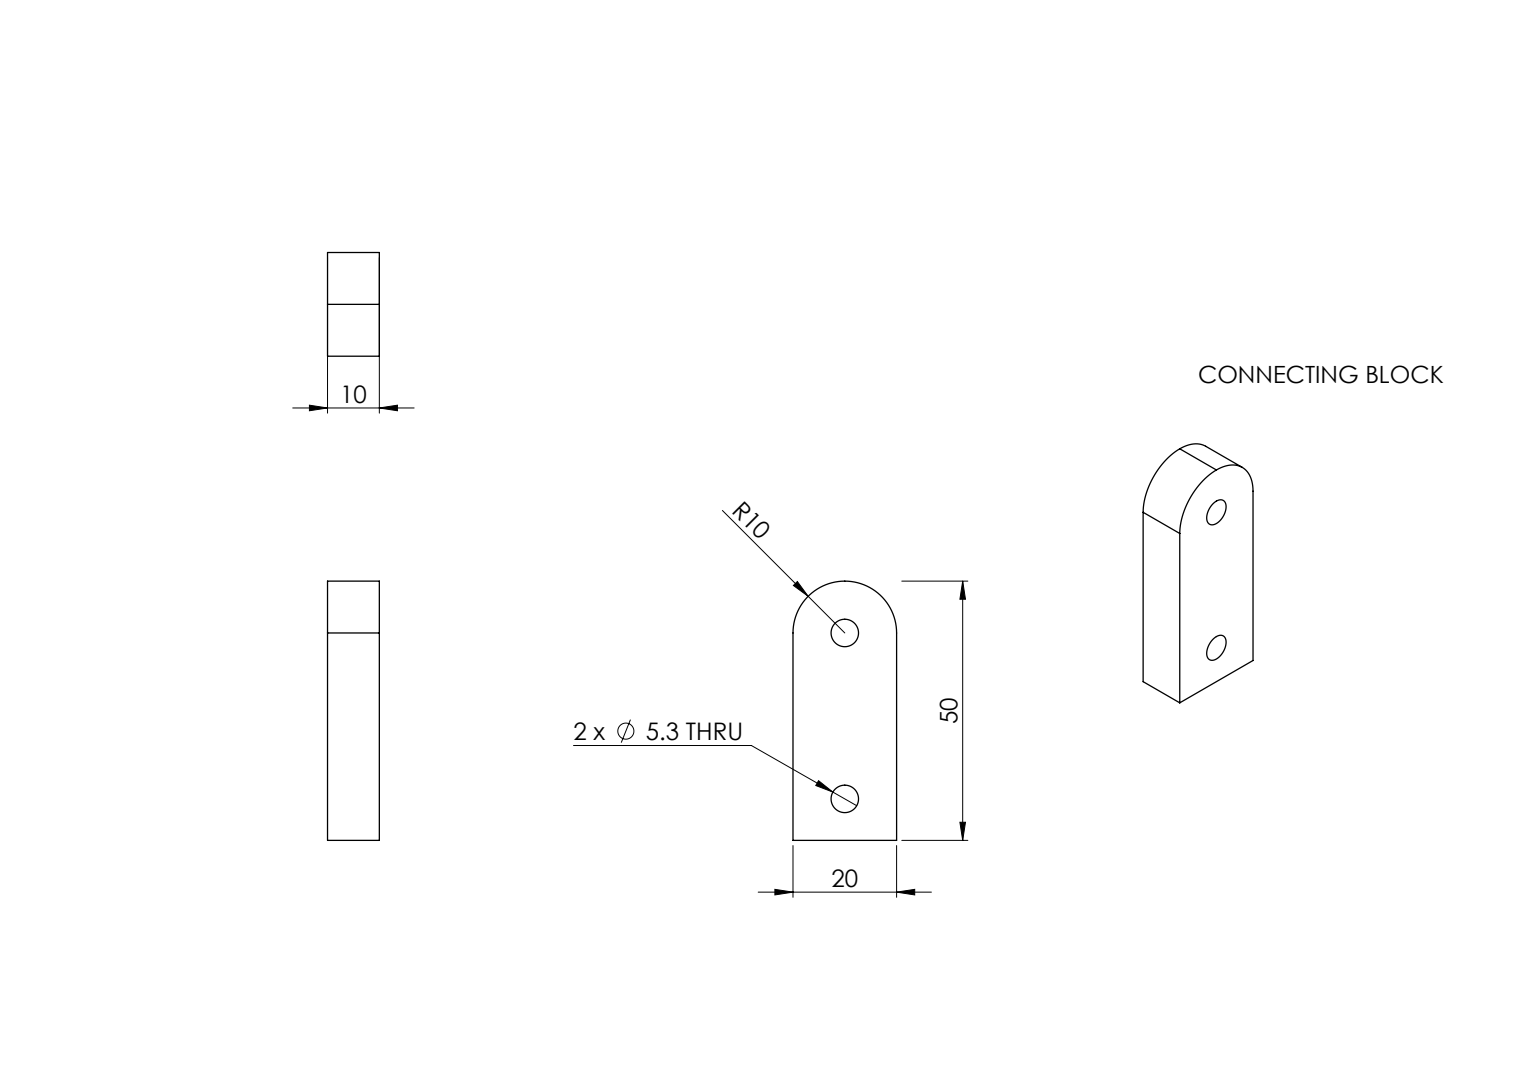
ISO-10303-21;
HEADER;
FILE_DESCRIPTION (('STEP AP214'),
    '1' );
FILE_NAME ('connecting block.step',
    '2026-10-25T17:17:34',
    ( '' ),
    ( '' ),
    'SwSTEP 2.0',
    'SolidWorks 2026',
    '' );
FILE_SCHEMA (( 'AUTOMOTIVE_DESIGN' ));
ENDSEC;

DATA;
#66=PLANE ( 'NONE',  #10236 ) ;
#158=DIRECTION ( 'NONE',  ( 0.000000000000000000, 1.000000000000000000, 0.000000000000000000 ) ) ;
#180=CARTESIAN_POINT ( 'NONE',  ( 109.9999999999999432, -29.80000000000002558, -150.0000000000000000 ) ) ;
#210=CARTESIAN_POINT ( 'NONE',  ( 99.99999999999994316, -29.80000000000000782, -150.0000000000000000 ) ) ;
#223=SHAPE_REPRESENTATION_RELATIONSHIP ( 'NONE' , 'NONE' ,  #14995, #14131 ) ;
#313=DIRECTION ( 'NONE',  ( 1.000000000000000000, -1.387778780781445676E-15, -2.407412430484046130E-31 ) ) ;
#489=CARTESIAN_POINT ( 'NONE',  ( 110.0000000000000142, 20.19999999999997797, -140.0000000000000000 ) ) ;
#517=ORIENTED_EDGE ( 'NONE', *, *, #5469, .F. ) ;
#541=CARTESIAN_POINT ( 'NONE',  ( 109.9999999999999574, -21.80000000000003268, -139.9999999999999716 ) ) ;
#670=ORIENTED_EDGE ( 'NONE', *, *, #8877, .T. ) ;
#820=AXIS2_PLACEMENT_3D ( 'NONE', #14217, #14502, #3869 ) ;
#918=DIRECTION ( 'NONE',  ( 1.000000000000000000, -0.000000000000000000, -2.407412430484046130E-31 ) ) ;
#945=EDGE_CURVE ( 'NONE', #2644, #11697, #6762, .T. ) ;
#972=ORIENTED_EDGE ( 'NONE', *, *, #12588, .F. ) ;
#1043=CLOSED_SHELL ( 'NONE', ( #15727, #1878, #15369, #14233, #4639, #15697, #12649, #17613, #16169, #5440, #19146 ) ) ;
#1064=ORIENTED_EDGE ( 'NONE', *, *, #3609, .F. ) ;
#1096=ORIENTED_EDGE ( 'NONE', *, *, #11672, .F. ) ;
#1137=CARTESIAN_POINT ( 'NONE',  ( 100.0000000000000000, 10.19999999999999396, -130.0000000000000000 ) ) ;
#1191=( GEOMETRIC_REPRESENTATION_CONTEXT ( 3 ) GLOBAL_UNCERTAINTY_ASSIGNED_CONTEXT ( ( #18445 ) ) GLOBAL_UNIT_ASSIGNED_CONTEXT ( ( #14859, #13397, #18984 ) ) REPRESENTATION_CONTEXT ( 'NONE', 'WORKASPACE' ) );
#1244=CARTESIAN_POINT ( 'NONE',  ( 110.0000000000000000, 10.19999999999997620, -139.9999999999999716 ) ) ;
#1398=ORIENTED_EDGE ( 'NONE', *, *, #4541, .F. ) ;
#1486=( NAMED_UNIT ( * ) PLANE_ANGLE_UNIT ( ) SI_UNIT ( $, .RADIAN. ) );
#1508=AXIS2_PLACEMENT_3D ( 'NONE', #9648, #2018, #10720 ) ;
#1521=ORIENTED_EDGE ( 'NONE', *, *, #7205, .T. ) ;
#1575=FACE_BOUND ( 'NONE', #12964, .T. ) ;
#1616=DIRECTION ( 'NONE',  ( 1.000000000000000000, -0.000000000000000000, -2.407412430484046130E-31 ) ) ;
#1660=ORIENTED_EDGE ( 'NONE', *, *, #11468, .T. ) ;
#1667=DIRECTION ( 'NONE',  ( -0.000000000000000000, 3.469446951953616161E-16, -1.000000000000000000 ) ) ;
#1747=CARTESIAN_POINT ( 'NONE',  ( 100.0000000000000000, 10.19999999999999218, -140.0000000000000000 ) ) ;
#1756=FACE_OUTER_BOUND ( 'NONE', #9533, .T. ) ;
#1775=EDGE_LOOP ( 'NONE', ( #3436, #14144, #6656, #3600 ) ) ;
#1829=ORIENTED_EDGE ( 'NONE', *, *, #5453, .T. ) ;
#1878=ADVANCED_FACE ( 'NONE', ( #10493 ), #15082, .F. ) ;
#1941=CARTESIAN_POINT ( 'NONE',  ( 100.0000000000000000, 10.19999999999997620, -142.6499999999999773 ) ) ;
#1993=ORIENTED_EDGE ( 'NONE', *, *, #4541, .T. ) ;
#2018=DIRECTION ( 'NONE',  ( 1.000000000000000000, -1.387778780781445676E-15, -2.407412430484046130E-31 ) ) ;
#2029=PRODUCT_CONTEXT ( 'NONE', #3323, 'mechanical' ) ;
#2039=EDGE_CURVE ( 'NONE', #3376, #2644, #2875, .T. ) ;
#2055=EDGE_LOOP ( 'NONE', ( #11819, #10542, #1398, #11442 ) ) ;
#2149=CARTESIAN_POINT ( 'NONE',  ( 110.0000000000000000, 10.19999999999997620, -150.0000000000000000 ) ) ;
#2320=EDGE_CURVE ( 'NONE', #17568, #9852, #15512, .T. ) ;
#2364=VECTOR ( 'NONE', #12931, 1000.000000000000000 ) ;
#2381=CARTESIAN_POINT ( 'NONE',  ( 110.0000000000000000, 10.19999999999997620, -139.9999999999999716 ) ) ;
#2411=CYLINDRICAL_SURFACE ( 'NONE', #16456, 10.00000000000000000 ) ;
#2569=DIRECTION ( 'NONE',  ( 1.000000000000000000, -1.387778780781445676E-15, -2.407412430484046130E-31 ) ) ;
#2628=ORIENTED_EDGE ( 'NONE', *, *, #2320, .F. ) ;
#2644=VERTEX_POINT ( 'NONE', #19175 ) ;
#2645=( NAMED_UNIT ( * ) SI_UNIT ( $, .STERADIAN. ) SOLID_ANGLE_UNIT ( ) );
#2685=LINE ( 'NONE', #9930, #9733 ) ;
#2706=LINE ( 'NONE', #180, #17740 ) ;
#2828=EDGE_CURVE ( 'NONE', #14354, #11020, #7827, .T. ) ;
#2875=LINE ( 'NONE', #6004, #5398 ) ;
#2934=DIRECTION ( 'NONE',  ( 1.000000000000000000, -1.387778780781445676E-15, -2.407412430484046130E-31 ) ) ;
#2998=DIRECTION ( 'NONE',  ( 0.000000000000000000, 1.000000000000000000, 0.000000000000000000 ) ) ;
#3041=CARTESIAN_POINT ( 'NONE',  ( 109.9999999999999432, -29.80000000000003268, -130.0000000000000000 ) ) ;
#3081=CYLINDRICAL_SURFACE ( 'NONE', #17126, 2.649999999999985700 ) ;
#3084=VERTEX_POINT ( 'NONE', #6227 ) ;
#3104=FACE_OUTER_BOUND ( 'NONE', #2055, .T. ) ;
#3218=CARTESIAN_POINT ( 'NONE',  ( 99.99999999999998579, -1.387778780781445676E-13, -2.407412430484045937E-29 ) ) ;
#3253=DIRECTION ( 'NONE',  ( -0.000000000000000000, 3.469446951953616161E-16, -1.000000000000000000 ) ) ;
#3323=APPLICATION_CONTEXT ( 'automotive_design' ) ;
#3325=DIRECTION ( 'NONE',  ( 0.000000000000000000, 1.000000000000000000, 0.000000000000000000 ) ) ;
#3359=CARTESIAN_POINT ( 'NONE',  ( 109.9999999999999432, -29.80000000000003268, -130.0000000000000000 ) ) ;
#3376=VERTEX_POINT ( 'NONE', #3041 ) ;
#3395=CARTESIAN_POINT ( 'NONE',  ( 109.9999999999999574, -21.80000000000003268, -137.3499999999999943 ) ) ;
#3429=ORIENTED_EDGE ( 'NONE', *, *, #16643, .F. ) ;
#3436=ORIENTED_EDGE ( 'NONE', *, *, #7205, .F. ) ;
#3474=ORIENTED_EDGE ( 'NONE', *, *, #2828, .T. ) ;
#3484=CARTESIAN_POINT ( 'NONE',  ( 99.99999999999994316, -29.80000000000000782, -150.0000000000000000 ) ) ;
#3507=AXIS2_PLACEMENT_3D ( 'NONE', #9368, #313, #6452 ) ;
#3600=ORIENTED_EDGE ( 'NONE', *, *, #4576, .F. ) ;
#3609=EDGE_CURVE ( 'NONE', #6906, #6376, #16464, .T. ) ;
#3618=VECTOR ( 'NONE', #8272, 1000.000000000000000 ) ;
#3669=CARTESIAN_POINT ( 'NONE',  ( 110.9999999999999574, -21.80000000000003268, -142.6499999999999773 ) ) ;
#3791=ORIENTED_EDGE ( 'NONE', *, *, #4723, .T. ) ;
#3869=DIRECTION ( 'NONE',  ( 1.387778780781445676E-15, 1.000000000000000000, -2.775557561562891351E-15 ) ) ;
#3999=AXIS2_PLACEMENT_3D ( 'NONE', #16398, #4385, #16215 ) ;
#4087=CARTESIAN_POINT ( 'NONE',  ( 100.0000000000000000, 10.19999999999997620, -139.9999999999999716 ) ) ;
#4203=LINE ( 'NONE', #10070, #8822 ) ;
#4346=DIRECTION ( 'NONE',  ( 1.000000000000000000, -0.000000000000000000, -2.407412430484046130E-31 ) ) ;
#4357=FACE_OUTER_BOUND ( 'NONE', #7999, .T. ) ;
#4375=CARTESIAN_POINT ( 'NONE',  ( 100.0000000000000000, 10.19999999999997620, -137.3499999999999943 ) ) ;
#4385=DIRECTION ( 'NONE',  ( -1.000000000000000000, 1.586032892321652482E-15, 0.000000000000000000 ) ) ;
#4413=PRESENTATION_STYLE_ASSIGNMENT (( #8611 ) ) ;
#4465=EDGE_CURVE ( 'NONE', #11020, #7039, #13361, .T. ) ;
#4538=ORIENTED_EDGE ( 'NONE', *, *, #8760, .F. ) ;
#4541=EDGE_CURVE ( 'NONE', #7039, #11136, #12486, .T. ) ;
#4542=CIRCLE ( 'NONE', #10784, 2.649999999999980371 ) ;
#4576=EDGE_CURVE ( 'NONE', #5794, #6376, #4790, .T. ) ;
#4639=ADVANCED_FACE ( 'NONE', ( #18652 ), #15907, .F. ) ;
#4653=DIRECTION ( 'NONE',  ( 0.000000000000000000, 0.000000000000000000, -1.000000000000000000 ) ) ;
#4723=EDGE_CURVE ( 'NONE', #2644, #7081, #2706, .T. ) ;
#4765=VECTOR ( 'NONE', #14074, 1000.000000000000000 ) ;
#4790=LINE ( 'NONE', #6442, #13665 ) ;
#4794=CIRCLE ( 'NONE', #7888, 9.999999999999998224 ) ;
#4841=CARTESIAN_POINT ( 'NONE',  ( 110.9999999999999574, -21.80000000000003268, -139.9999999999999716 ) ) ;
#4895=DIRECTION ( 'NONE',  ( 1.387778780781445873E-15, 1.000000000000000000, 0.000000000000000000 ) ) ;
#4936=LINE ( 'NONE', #3359, #5998 ) ;
#4993=CARTESIAN_POINT ( 'NONE',  ( 100.0000000000000000, 10.19999999999997620, -139.9999999999999716 ) ) ;
#5099=EDGE_LOOP ( 'NONE', ( #4538, #17421, #7613, #1660 ) ) ;
#5232=AXIS2_PLACEMENT_3D ( 'NONE', #6966, #9796, #18700 ) ;
#5276=VERTEX_POINT ( 'NONE', #10120 ) ;
#5316=FACE_OUTER_BOUND ( 'NONE', #1775, .T. ) ;
#5398=VECTOR ( 'NONE', #3253, 1000.000000000000000 ) ;
#5440=ADVANCED_FACE ( 'NONE', ( #12445 ), #16746, .F. ) ;
#5453=EDGE_CURVE ( 'NONE', #8145, #9264, #12430, .T. ) ;
#5469=EDGE_CURVE ( 'NONE', #14354, #3376, #4936, .T. ) ;
#5508=FACE_OUTER_BOUND ( 'NONE', #8430, .T. ) ;
#5560=( GEOMETRIC_REPRESENTATION_CONTEXT ( 3 ) GLOBAL_UNCERTAINTY_ASSIGNED_CONTEXT ( ( #13232 ) ) GLOBAL_UNIT_ASSIGNED_CONTEXT ( ( #17901, #1486, #2645 ) ) REPRESENTATION_CONTEXT ( 'NONE', 'WORKASPACE' ) );
#5570=AXIS2_PLACEMENT_3D ( 'NONE', #17281, #9661, #12969 ) ;
#5577=CIRCLE ( 'NONE', #1508, 9.999999999999998224 ) ;
#5683=CARTESIAN_POINT ( 'NONE',  ( 111.0000000000000000, 10.19999999999997620, -137.3499999999999943 ) ) ;
#5736=DIRECTION ( 'NONE',  ( -0.000000000000000000, 0.000000000000000000, 1.000000000000000000 ) ) ;
#5768=DIRECTION ( 'NONE',  ( 1.000000000000000000, -0.000000000000000000, -2.407412430484046130E-31 ) ) ;
#5784=FILL_AREA_STYLE ('',( #17803 ) ) ;
#5794=VERTEX_POINT ( 'NONE', #1941 ) ;
#5899=DIRECTION ( 'NONE',  ( 1.000000000000000000, -1.387778780781445676E-15, -2.407412430484046130E-31 ) ) ;
#5998=VECTOR ( 'NONE', #16851, 1000.000000000000000 ) ;
#6004=CARTESIAN_POINT ( 'NONE',  ( 109.9999999999999432, -29.80000000000002558, -150.0000000000000000 ) ) ;
#6010=CIRCLE ( 'NONE', #3507, 2.649999999999982148 ) ;
#6028=VECTOR ( 'NONE', #5768, 1000.000000000000000 ) ;
#6188=VERTEX_POINT ( 'NONE', #4375 ) ;
#6227=CARTESIAN_POINT ( 'NONE',  ( 100.0000000000000000, 10.19999999999999396, -150.0000000000000000 ) ) ;
#6359=CARTESIAN_POINT ( 'NONE',  ( 110.0000000000000000, 10.19999999999997620, -139.9999999999999716 ) ) ;
#6369=EDGE_LOOP ( 'NONE', ( #17719, #15739, #15622, #12797 ) ) ;
#6370=DIRECTION ( 'NONE',  ( -1.000000000000000000, 1.586032892321652482E-15, 0.000000000000000000 ) ) ;
#6376=VERTEX_POINT ( 'NONE', #16677 ) ;
#6442=CARTESIAN_POINT ( 'NONE',  ( 111.0000000000000000, 10.19999999999997620, -142.6499999999999773 ) ) ;
#6452=DIRECTION ( 'NONE',  ( 0.000000000000000000, 1.000000000000000000, 0.000000000000000000 ) ) ;
#6616=EDGE_CURVE ( 'NONE', #11697, #3084, #2685, .T. ) ;
#6648=CARTESIAN_POINT ( 'NONE',  ( 100.0000000000000142, 20.19999999999999574, -140.0000000000000000 ) ) ;
#6656=ORIENTED_EDGE ( 'NONE', *, *, #3609, .T. ) ;
#6659=DIRECTION ( 'NONE',  ( 1.000000000000000000, -1.387778780781445676E-15, -2.407412430484046130E-31 ) ) ;
#6681=PLANE ( 'NONE',  #5232 ) ;
#6762=LINE ( 'NONE', #15839, #4765 ) ;
#6802=COLOUR_RGB ( '',0.8941176470588234615, 0.8941176470588234615, 0.8941176470588234615 ) ;
#6906=VERTEX_POINT ( 'NONE', #19184 ) ;
#6966=CARTESIAN_POINT ( 'NONE',  ( 109.9999999999999858, -1.546382070013610932E-13, -2.407412430484045937E-29 ) ) ;
#7013=EDGE_CURVE ( 'NONE', #9852, #17568, #6010, .T. ) ;
#7039=VERTEX_POINT ( 'NONE', #6648 ) ;
#7081=VERTEX_POINT ( 'NONE', #2149 ) ;
#7106=ORIENTED_EDGE ( 'NONE', *, *, #11374, .F. ) ;
#7111=STYLED_ITEM ( 'NONE', ( #4413 ), #14131 ) ;
#7205=EDGE_CURVE ( 'NONE', #6188, #5794, #10689, .T. ) ;
#7262=AXIS2_PLACEMENT_3D ( 'NONE', #4993, #10936, #15431 ) ;
#7264=CARTESIAN_POINT ( 'NONE',  ( 110.0000000000000000, 10.19999999999997620, -130.0000000000000000 ) ) ;
#7327=ORIENTED_EDGE ( 'NONE', *, *, #2039, .T. ) ;
#7341=CARTESIAN_POINT ( 'NONE',  ( 0.000000000000000000, 0.000000000000000000, 0.000000000000000000 ) ) ;
#7516=MANIFOLD_SOLID_BREP ( 'M5 Clearance Hole1', #1043 ) ;
#7523=DIRECTION ( 'NONE',  ( 1.387778780781445676E-15, 1.000000000000000000, 0.000000000000000000 ) ) ;
#7578=DIRECTION ( 'NONE',  ( 0.000000000000000000, 0.000000000000000000, -1.000000000000000000 ) ) ;
#7613=ORIENTED_EDGE ( 'NONE', *, *, #4576, .T. ) ;
#7827=LINE ( 'NONE', #13782, #8641 ) ;
#7888=AXIS2_PLACEMENT_3D ( 'NONE', #6359, #15634, #4895 ) ;
#7932=EDGE_CURVE ( 'NONE', #7081, #11136, #4794, .T. ) ;
#7999=EDGE_LOOP ( 'NONE', ( #517, #3474, #11002, #14020 ) ) ;
#8145=VERTEX_POINT ( 'NONE', #3395 ) ;
#8272=DIRECTION ( 'NONE',  ( 1.000000000000000000, -1.586032892321652482E-15, 0.000000000000000000 ) ) ;
#8359=EDGE_LOOP ( 'NONE', ( #2628, #12481, #1829, #3429 ) ) ;
#8430=EDGE_LOOP ( 'NONE', ( #3791, #12729, #15733, #8546, #7327 ) ) ;
#8435=CARTESIAN_POINT ( 'NONE',  ( 110.9999999999999574, -21.80000000000003268, -137.3499999999999943 ) ) ;
#8463=FACE_OUTER_BOUND ( 'NONE', #12711, .T. ) ;
#8546=ORIENTED_EDGE ( 'NONE', *, *, #5469, .T. ) ;
#8593=ORIENTED_EDGE ( 'NONE', *, *, #7013, .T. ) ;
#8611=SURFACE_STYLE_USAGE ( .BOTH. , #10281 ) ;
#8641=VECTOR ( 'NONE', #6370, 1000.000000000000000 ) ;
#8654=CARTESIAN_POINT ( 'NONE',  ( 111.0000000000000000, 10.19999999999997620, -139.9999999999999716 ) ) ;
#8696=LINE ( 'NONE', #5683, #6028 ) ;
#8760=EDGE_CURVE ( 'NONE', #6188, #6906, #8696, .T. ) ;
#8817=CARTESIAN_POINT ( 'NONE',  ( 109.9999999999999574, -21.80000000000003268, -139.9999999999999716 ) ) ;
#8822=VECTOR ( 'NONE', #13277, 1000.000000000000000 ) ;
#8877=EDGE_CURVE ( 'NONE', #3376, #5276, #4203, .T. ) ;
#9040=DIRECTION ( 'NONE',  ( 1.000000000000000000, 0.000000000000000000, 0.000000000000000000 ) ) ;
#9098=EDGE_CURVE ( 'NONE', #9264, #8145, #10085, .T. ) ;
#9264=VERTEX_POINT ( 'NONE', #9488 ) ;
#9368=CARTESIAN_POINT ( 'NONE',  ( 99.99999999999995737, -21.80000000000003268, -139.9999999999999716 ) ) ;
#9480=ORIENTED_EDGE ( 'NONE', *, *, #2039, .F. ) ;
#9488=CARTESIAN_POINT ( 'NONE',  ( 109.9999999999999574, -21.80000000000003268, -142.6499999999999773 ) ) ;
#9533=EDGE_LOOP ( 'NONE', ( #16683, #13175, #14475, #972, #9819 ) ) ;
#9648=CARTESIAN_POINT ( 'NONE',  ( 110.0000000000000000, 10.19999999999997620, -140.0000000000000000 ) ) ;
#9661=DIRECTION ( 'NONE',  ( 1.586032892321652482E-15, 1.000000000000000000, 3.469446951953616654E-16 ) ) ;
#9733=VECTOR ( 'NONE', #11489, 1000.000000000000000 ) ;
#9796=DIRECTION ( 'NONE',  ( 1.000000000000000000, -1.387778780781445676E-15, -2.407412430484046130E-31 ) ) ;
#9819=ORIENTED_EDGE ( 'NONE', *, *, #15245, .F. ) ;
#9852=VERTEX_POINT ( 'NONE', #16105 ) ;
#9884=EDGE_CURVE ( 'NONE', #5794, #6188, #16382, .T. ) ;
#9930=CARTESIAN_POINT ( 'NONE',  ( 99.99999999999994316, -29.80000000000000782, -150.0000000000000000 ) ) ;
#9934=AXIS2_PLACEMENT_3D ( 'NONE', #1747, #15229, #15321 ) ;
#9988=( NAMED_UNIT ( * ) PLANE_ANGLE_UNIT ( ) SI_UNIT ( $, .RADIAN. ) );
#10033=CARTESIAN_POINT ( 'NONE',  ( 99.99999999999994316, -29.80000000000001492, -130.0000000000000000 ) ) ;
#10070=CARTESIAN_POINT ( 'NONE',  ( 109.9999999999999432, -29.80000000000003268, -130.0000000000000000 ) ) ;
#10085=CIRCLE ( 'NONE', #12573, 2.649999999999982148 ) ;
#10120=CARTESIAN_POINT ( 'NONE',  ( 99.99999999999994316, -29.80000000000001492, -130.0000000000000000 ) ) ;
#10130=FACE_OUTER_BOUND ( 'NONE', #6369, .T. ) ;
#10156=ORIENTED_EDGE ( 'NONE', *, *, #9098, .F. ) ;
#10236=AXIS2_PLACEMENT_3D ( 'NONE', #15001, #4653, #16471 ) ;
#10281=SURFACE_SIDE_STYLE ('',( #17705 ) ) ;
#10359=LINE ( 'NONE', #210, #18915 ) ;
#10373=MECHANICAL_DESIGN_GEOMETRIC_PRESENTATION_REPRESENTATION('',(#18805),#17871);
#10476=DIRECTION ( 'NONE',  ( 0.000000000000000000, 1.000000000000000000, 0.000000000000000000 ) ) ;
#10493=FACE_OUTER_BOUND ( 'NONE', #8359, .T. ) ;
#10509=FACE_OUTER_BOUND ( 'NONE', #5099, .T. ) ;
#10514=AXIS2_PLACEMENT_3D ( 'NONE', #14565, #17609, #17228 ) ;
#10529=AXIS2_PLACEMENT_3D ( 'NONE', #11135, #6659, #3325 ) ;
#10540=AXIS2_PLACEMENT_3D ( 'NONE', #7341, #19270, #11738 ) ;
#10542=ORIENTED_EDGE ( 'NONE', *, *, #13895, .F. ) ;
#10689=CIRCLE ( 'NONE', #7262, 2.649999999999980371 ) ;
#10720=DIRECTION ( 'NONE',  ( 1.387778780781445873E-15, 1.000000000000000000, 0.000000000000000000 ) ) ;
#10784=AXIS2_PLACEMENT_3D ( 'NONE', #2381, #2569, #11270 ) ;
#10900=EDGE_CURVE ( 'NONE', #7039, #3084, #18287, .T. ) ;
#10936=DIRECTION ( 'NONE',  ( 1.000000000000000000, -1.387778780781445676E-15, -2.407412430484046130E-31 ) ) ;
#11002=ORIENTED_EDGE ( 'NONE', *, *, #15245, .T. ) ;
#11020=VERTEX_POINT ( 'NONE', #1137 ) ;
#11030=AXIS2_PLACEMENT_3D ( 'NONE', #4841, #1616, #13903 ) ;
#11086=LINE ( 'NONE', #3669, #16786 ) ;
#11135=CARTESIAN_POINT ( 'NONE',  ( 110.0000000000000000, 10.19999999999997620, -139.9999999999999716 ) ) ;
#11136=VERTEX_POINT ( 'NONE', #16370 ) ;
#11270=DIRECTION ( 'NONE',  ( 0.000000000000000000, 1.000000000000000000, 0.000000000000000000 ) ) ;
#11355=FACE_BOUND ( 'NONE', #15638, .T. ) ;
#11374=EDGE_CURVE ( 'NONE', #17568, #8145, #17241, .T. ) ;
#11442=ORIENTED_EDGE ( 'NONE', *, *, #4465, .F. ) ;
#11468=EDGE_CURVE ( 'NONE', #6376, #6906, #4542, .T. ) ;
#11489=DIRECTION ( 'NONE',  ( 1.387778780781445676E-15, 1.000000000000000000, 0.000000000000000000 ) ) ;
#11550=DIRECTION ( 'NONE',  ( 0.000000000000000000, 0.000000000000000000, -1.000000000000000000 ) ) ;
#11590=PLANE ( 'NONE',  #13007 ) ;
#11593=DIRECTION ( 'NONE',  ( -1.387778780781445676E-15, -1.000000000000000000, 0.000000000000000000 ) ) ;
#11672=EDGE_CURVE ( 'NONE', #3084, #7081, #12663, .T. ) ;
#11697=VERTEX_POINT ( 'NONE', #3484 ) ;
#11738=DIRECTION ( 'NONE',  ( 1.000000000000000000, 0.000000000000000000, 0.000000000000000000 ) ) ;
#11819=ORIENTED_EDGE ( 'NONE', *, *, #2828, .F. ) ;
#12082=AXIS2_PLACEMENT_3D ( 'NONE', #13012, #918, #11550 ) ;
#12128=ORIENTED_EDGE ( 'NONE', *, *, #7013, .F. ) ;
#12137=EDGE_LOOP ( 'NONE', ( #16984, #1521 ) ) ;
#12366=ORIENTED_EDGE ( 'NONE', *, *, #2320, .T. ) ;
#12394=DIRECTION ( 'NONE',  ( 1.000000000000000000, -0.000000000000000000, -2.407412430484046130E-31 ) ) ;
#12430=CIRCLE ( 'NONE', #18482, 2.649999999999982148 ) ;
#12445=FACE_OUTER_BOUND ( 'NONE', #13778, .T. ) ;
#12481=ORIENTED_EDGE ( 'NONE', *, *, #11374, .T. ) ;
#12486=LINE ( 'NONE', #489, #18979 ) ;
#12573=AXIS2_PLACEMENT_3D ( 'NONE', #8817, #5899, #10476 ) ;
#12580=SHAPE_DEFINITION_REPRESENTATION ( #18730, #14995 ) ;
#12588=EDGE_CURVE ( 'NONE', #5276, #11697, #10359, .T. ) ;
#12649=ADVANCED_FACE ( 'NONE', ( #15139, #1575, #1756 ), #16611, .F. ) ;
#12663=LINE ( 'NONE', #18636, #3618 ) ;
#12711=EDGE_LOOP ( 'NONE', ( #15599, #1096, #16031, #1993 ) ) ;
#12729=ORIENTED_EDGE ( 'NONE', *, *, #7932, .T. ) ;
#12793=PRODUCT ( 'connecting block', 'connecting block', '', ( #2029 ) ) ;
#12797=ORIENTED_EDGE ( 'NONE', *, *, #945, .T. ) ;
#12806=ORIENTED_EDGE ( 'NONE', *, *, #12588, .T. ) ;
#12868=DIRECTION ( 'NONE',  ( -1.000000000000000000, 1.586032892321652482E-15, 0.000000000000000000 ) ) ;
#12931=DIRECTION ( 'NONE',  ( 1.000000000000000000, -0.000000000000000000, -2.407412430484046130E-31 ) ) ;
#12964=EDGE_LOOP ( 'NONE', ( #8593, #12366 ) ) ;
#12969=DIRECTION ( 'NONE',  ( -1.000000000000000000, 1.586032892321652482E-15, 0.000000000000000000 ) ) ;
#13007=AXIS2_PLACEMENT_3D ( 'NONE', #17555, #5736, #9040 ) ;
#13012=CARTESIAN_POINT ( 'NONE',  ( 111.0000000000000000, 10.19999999999997620, -139.9999999999999716 ) ) ;
#13105=ORIENTED_EDGE ( 'NONE', *, *, #945, .F. ) ;
#13160=DIRECTION ( 'NONE',  ( 1.000000000000000000, -1.387778780781445676E-15, -2.407412430484046130E-31 ) ) ;
#13175=ORIENTED_EDGE ( 'NONE', *, *, #10900, .T. ) ;
#13232=UNCERTAINTY_MEASURE_WITH_UNIT (LENGTH_MEASURE( 1.000000000000000082E-05 ), #17901, 'distance_accuracy_value', 'NONE');
#13277=DIRECTION ( 'NONE',  ( -1.000000000000000000, 1.586032892321652482E-15, -0.000000000000000000 ) ) ;
#13346=DIRECTION ( 'NONE',  ( 1.000000000000000000, -0.000000000000000000, -2.407412430484046130E-31 ) ) ;
#13361=CIRCLE ( 'NONE', #9934, 10.00000000000000000 ) ;
#13397=( NAMED_UNIT ( * ) PLANE_ANGLE_UNIT ( ) SI_UNIT ( $, .RADIAN. ) );
#13665=VECTOR ( 'NONE', #12394, 1000.000000000000000 ) ;
#13778=EDGE_LOOP ( 'NONE', ( #7106, #12128, #18212, #16093 ) ) ;
#13782=CARTESIAN_POINT ( 'NONE',  ( 110.0000000000000142, 10.19999999999997620, -130.0000000000000000 ) ) ;
#13895=EDGE_CURVE ( 'NONE', #11136, #14354, #5577, .T. ) ;
#13903=DIRECTION ( 'NONE',  ( 0.000000000000000000, 0.000000000000000000, -1.000000000000000000 ) ) ;
#14020=ORIENTED_EDGE ( 'NONE', *, *, #8877, .F. ) ;
#14074=DIRECTION ( 'NONE',  ( -1.000000000000000000, 1.586032892321652482E-15, -0.000000000000000000 ) ) ;
#14131=ADVANCED_BREP_SHAPE_REPRESENTATION ( '', ( #7516, #10540 ), #5560 ) ;
#14144=ORIENTED_EDGE ( 'NONE', *, *, #8760, .T. ) ;
#14217=CARTESIAN_POINT ( 'NONE',  ( 100.0000000000000000, 10.19999999999999218, -139.9999999999999716 ) ) ;
#14233=ADVANCED_FACE ( 'NONE', ( #4357 ), #66, .F. ) ;
#14249=PRODUCT_DEFINITION_FORMATION_WITH_SPECIFIED_SOURCE ( 'ANY', '', #12793, .NOT_KNOWN. ) ;
#14266=ORIENTED_EDGE ( 'NONE', *, *, #11468, .F. ) ;
#14354=VERTEX_POINT ( 'NONE', #7264 ) ;
#14463=CYLINDRICAL_SURFACE ( 'NONE', #12082, 2.649999999999985700 ) ;
#14475=ORIENTED_EDGE ( 'NONE', *, *, #6616, .F. ) ;
#14502=DIRECTION ( 'NONE',  ( -1.000000000000000000, 1.387778780781445676E-15, 2.407412430484046130E-31 ) ) ;
#14565=CARTESIAN_POINT ( 'NONE',  ( 99.99999999999995737, -21.80000000000003268, -139.9999999999999716 ) ) ;
#14859=( LENGTH_UNIT ( ) NAMED_UNIT ( * ) SI_UNIT ( .MILLI., .METRE. ) );
#14995=SHAPE_REPRESENTATION ( 'connecting block', ( #10540 ), #5560 ) ;
#15001=CARTESIAN_POINT ( 'NONE',  ( 109.9999999999999432, -29.80000000000003268, -130.0000000000000000 ) ) ;
#15082=CYLINDRICAL_SURFACE ( 'NONE', #15678, 2.649999999999985700 ) ;
#15139=FACE_BOUND ( 'NONE', #12137, .T. ) ;
#15229=DIRECTION ( 'NONE',  ( -1.000000000000000000, 1.387778780781445676E-15, 2.407412430484046130E-31 ) ) ;
#15245=EDGE_CURVE ( 'NONE', #11020, #5276, #15708, .T. ) ;
#15291=PRODUCT_DEFINITION_CONTEXT ( 'detailed design', #18573, 'design' ) ;
#15321=DIRECTION ( 'NONE',  ( 1.387778780781445676E-15, 1.000000000000000000, 0.000000000000000000 ) ) ;
#15352=EDGE_LOOP ( 'NONE', ( #12806, #13105, #9480, #670 ) ) ;
#15369=ADVANCED_FACE ( 'NONE', ( #10130 ), #11590, .F. ) ;
#15431=DIRECTION ( 'NONE',  ( 0.000000000000000000, 1.000000000000000000, 0.000000000000000000 ) ) ;
#15512=CIRCLE ( 'NONE', #10514, 2.649999999999982148 ) ;
#15537=MECHANICAL_DESIGN_GEOMETRIC_PRESENTATION_REPRESENTATION('',(#7111),#1191);
#15599=ORIENTED_EDGE ( 'NONE', *, *, #7932, .F. ) ;
#15622=ORIENTED_EDGE ( 'NONE', *, *, #4723, .F. ) ;
#15634=DIRECTION ( 'NONE',  ( 1.000000000000000000, -1.387778780781445676E-15, -2.407412430484046130E-31 ) ) ;
#15638=EDGE_LOOP ( 'NONE', ( #14266, #1064 ) ) ;
#15678=AXIS2_PLACEMENT_3D ( 'NONE', #16264, #4346, #16650 ) ;
#15697=ADVANCED_FACE ( 'NONE', ( #11355, #17129, #5508 ), #6681, .T. ) ;
#15708=LINE ( 'NONE', #10033, #17391 ) ;
#15727=ADVANCED_FACE ( 'NONE', ( #5316 ), #14463, .F. ) ;
#15733=ORIENTED_EDGE ( 'NONE', *, *, #13895, .T. ) ;
#15739=ORIENTED_EDGE ( 'NONE', *, *, #11672, .T. ) ;
#15785=UNCERTAINTY_MEASURE_WITH_UNIT (LENGTH_MEASURE( 1.000000000000000082E-05 ), #16137, 'distance_accuracy_value', 'NONE');
#15790=EDGE_LOOP ( 'NONE', ( #10156, #17617 ) ) ;
#15803=DIRECTION ( 'NONE',  ( -1.387778780781445676E-15, -1.000000000000000000, -0.000000000000000000 ) ) ;
#15839=CARTESIAN_POINT ( 'NONE',  ( 109.9999999999999432, -29.80000000000002558, -150.0000000000000000 ) ) ;
#15861=PRODUCT_DEFINITION ( 'UNKNOWN', '', #14249, #15291 ) ;
#15907=PLANE ( 'NONE',  #5570 ) ;
#15943=( NAMED_UNIT ( * ) SI_UNIT ( $, .STERADIAN. ) SOLID_ANGLE_UNIT ( ) );
#16031=ORIENTED_EDGE ( 'NONE', *, *, #10900, .F. ) ;
#16093=ORIENTED_EDGE ( 'NONE', *, *, #9098, .T. ) ;
#16105=CARTESIAN_POINT ( 'NONE',  ( 99.99999999999995737, -21.80000000000003268, -142.6499999999999773 ) ) ;
#16137=( LENGTH_UNIT ( ) NAMED_UNIT ( * ) SI_UNIT ( .MILLI., .METRE. ) );
#16169=ADVANCED_FACE ( 'NONE', ( #8463 ), #2411, .T. ) ;
#16215=DIRECTION ( 'NONE',  ( -1.387778780781445676E-15, -1.000000000000000000, 0.000000000000000000 ) ) ;
#16264=CARTESIAN_POINT ( 'NONE',  ( 110.9999999999999574, -21.80000000000003268, -139.9999999999999716 ) ) ;
#16306=CARTESIAN_POINT ( 'NONE',  ( 99.99999999999995737, -21.80000000000003268, -137.3499999999999943 ) ) ;
#16370=CARTESIAN_POINT ( 'NONE',  ( 110.0000000000000142, 20.19999999999997797, -140.0000000000000000 ) ) ;
#16382=CIRCLE ( 'NONE', #18890, 2.649999999999980371 ) ;
#16398=CARTESIAN_POINT ( 'NONE',  ( 110.0000000000000142, 10.19999999999997620, -140.0000000000000000 ) ) ;
#16456=AXIS2_PLACEMENT_3D ( 'NONE', #1244, #12868, #11593 ) ;
#16464=CIRCLE ( 'NONE', #10529, 2.649999999999980371 ) ;
#16471=DIRECTION ( 'NONE',  ( -1.000000000000000000, 0.000000000000000000, -0.000000000000000000 ) ) ;
#16611=PLANE ( 'NONE',  #16732 ) ;
#16643=EDGE_CURVE ( 'NONE', #9852, #9264, #11086, .T. ) ;
#16650=DIRECTION ( 'NONE',  ( 0.000000000000000000, 0.000000000000000000, -1.000000000000000000 ) ) ;
#16677=CARTESIAN_POINT ( 'NONE',  ( 110.0000000000000000, 10.19999999999997620, -142.6499999999999773 ) ) ;
#16683=ORIENTED_EDGE ( 'NONE', *, *, #4465, .T. ) ;
#16732=AXIS2_PLACEMENT_3D ( 'NONE', #3218, #2934, #7523 ) ;
#16746=CYLINDRICAL_SURFACE ( 'NONE', #11030, 2.649999999999985700 ) ;
#16786=VECTOR ( 'NONE', #16864, 1000.000000000000000 ) ;
#16851=DIRECTION ( 'NONE',  ( -1.387778780781445676E-15, -1.000000000000000000, -0.000000000000000000 ) ) ;
#16864=DIRECTION ( 'NONE',  ( 1.000000000000000000, -0.000000000000000000, -2.407412430484046130E-31 ) ) ;
#16984=ORIENTED_EDGE ( 'NONE', *, *, #9884, .T. ) ;
#17126=AXIS2_PLACEMENT_3D ( 'NONE', #8654, #13346, #7578 ) ;
#17129=FACE_BOUND ( 'NONE', #15790, .T. ) ;
#17228=DIRECTION ( 'NONE',  ( 0.000000000000000000, 1.000000000000000000, 0.000000000000000000 ) ) ;
#17241=LINE ( 'NONE', #8435, #2364 ) ;
#17281=CARTESIAN_POINT ( 'NONE',  ( 109.9999999999999432, -29.80000000000002558, -150.0000000000000000 ) ) ;
#17391=VECTOR ( 'NONE', #15803, 1000.000000000000000 ) ;
#17421=ORIENTED_EDGE ( 'NONE', *, *, #9884, .F. ) ;
#17555=CARTESIAN_POINT ( 'NONE',  ( 109.9999999999999432, -29.80000000000002558, -150.0000000000000000 ) ) ;
#17568=VERTEX_POINT ( 'NONE', #16306 ) ;
#17609=DIRECTION ( 'NONE',  ( 1.000000000000000000, -1.387778780781445676E-15, -2.407412430484046130E-31 ) ) ;
#17613=ADVANCED_FACE ( 'NONE', ( #3104 ), #17965, .T. ) ;
#17617=ORIENTED_EDGE ( 'NONE', *, *, #5453, .F. ) ;
#17705=SURFACE_STYLE_FILL_AREA ( #5784 ) ;
#17719=ORIENTED_EDGE ( 'NONE', *, *, #6616, .T. ) ;
#17740=VECTOR ( 'NONE', #17764, 1000.000000000000000 ) ;
#17764=DIRECTION ( 'NONE',  ( 1.387778780781445676E-15, 1.000000000000000000, 0.000000000000000000 ) ) ;
#17803=FILL_AREA_STYLE_COLOUR ( '', #6802 ) ;
#17871=( GEOMETRIC_REPRESENTATION_CONTEXT ( 3 ) GLOBAL_UNCERTAINTY_ASSIGNED_CONTEXT ( ( #15785 ) ) GLOBAL_UNIT_ASSIGNED_CONTEXT ( ( #16137, #9988, #15943 ) ) REPRESENTATION_CONTEXT ( 'NONE', 'WORKASPACE' ) );
#17901=( LENGTH_UNIT ( ) NAMED_UNIT ( * ) SI_UNIT ( .MILLI., .METRE. ) );
#17965=CYLINDRICAL_SURFACE ( 'NONE', #3999, 10.00000000000000000 ) ;
#18212=ORIENTED_EDGE ( 'NONE', *, *, #16643, .T. ) ;
#18287=CIRCLE ( 'NONE', #820, 10.00000000000000000 ) ;
#18413=DIRECTION ( 'NONE',  ( 1.000000000000000000, -1.387778780781445676E-15, -2.407412430484046130E-31 ) ) ;
#18445=UNCERTAINTY_MEASURE_WITH_UNIT (LENGTH_MEASURE( 1.000000000000000082E-05 ), #14859, 'distance_accuracy_value', 'NONE');
#18482=AXIS2_PLACEMENT_3D ( 'NONE', #541, #18413, #158 ) ;
#18552=DIRECTION ( 'NONE',  ( 1.000000000000000000, -1.586032892321652482E-15, -0.000000000000000000 ) ) ;
#18573=APPLICATION_CONTEXT ( 'automotive_design' ) ;
#18636=CARTESIAN_POINT ( 'NONE',  ( 110.0000000000000142, 10.19999999999997620, -150.0000000000000000 ) ) ;
#18652=FACE_OUTER_BOUND ( 'NONE', #15352, .T. ) ;
#18700=DIRECTION ( 'NONE',  ( 1.387778780781445676E-15, 1.000000000000000000, 0.000000000000000000 ) ) ;
#18730=PRODUCT_DEFINITION_SHAPE ( 'NONE', 'NONE',  #15861 ) ;
#18805=STYLED_ITEM('',(#19343),#7516);
#18890=AXIS2_PLACEMENT_3D ( 'NONE', #4087, #13160, #2998 ) ;
#18915=VECTOR ( 'NONE', #1667, 1000.000000000000000 ) ;
#18979=VECTOR ( 'NONE', #18552, 1000.000000000000000 ) ;
#18984=( NAMED_UNIT ( * ) SI_UNIT ( $, .STERADIAN. ) SOLID_ANGLE_UNIT ( ) );
#19146=ADVANCED_FACE ( 'NONE', ( #10509 ), #3081, .F. ) ;
#19175=CARTESIAN_POINT ( 'NONE',  ( 109.9999999999999432, -29.80000000000002558, -150.0000000000000000 ) ) ;
#19184=CARTESIAN_POINT ( 'NONE',  ( 110.0000000000000000, 10.19999999999997620, -137.3499999999999943 ) ) ;
#19270=DIRECTION ( 'NONE',  ( 0.000000000000000000, 0.000000000000000000, 1.000000000000000000 ) ) ;
#19337=COLOUR_RGB('Dark Blue',0.08,0.2,0.34);
#19338=FILL_AREA_STYLE_COLOUR('',#19337);
#19339=FILL_AREA_STYLE('',(#19338));
#19340=SURFACE_STYLE_FILL_AREA(#19339);
#19341=SURFACE_SIDE_STYLE('',(#19340));
#19342=SURFACE_STYLE_USAGE(.BOTH.,#19341);
#19343=PRESENTATION_STYLE_ASSIGNMENT((#19342));
ENDSEC;
END-ISO-10303-21;
